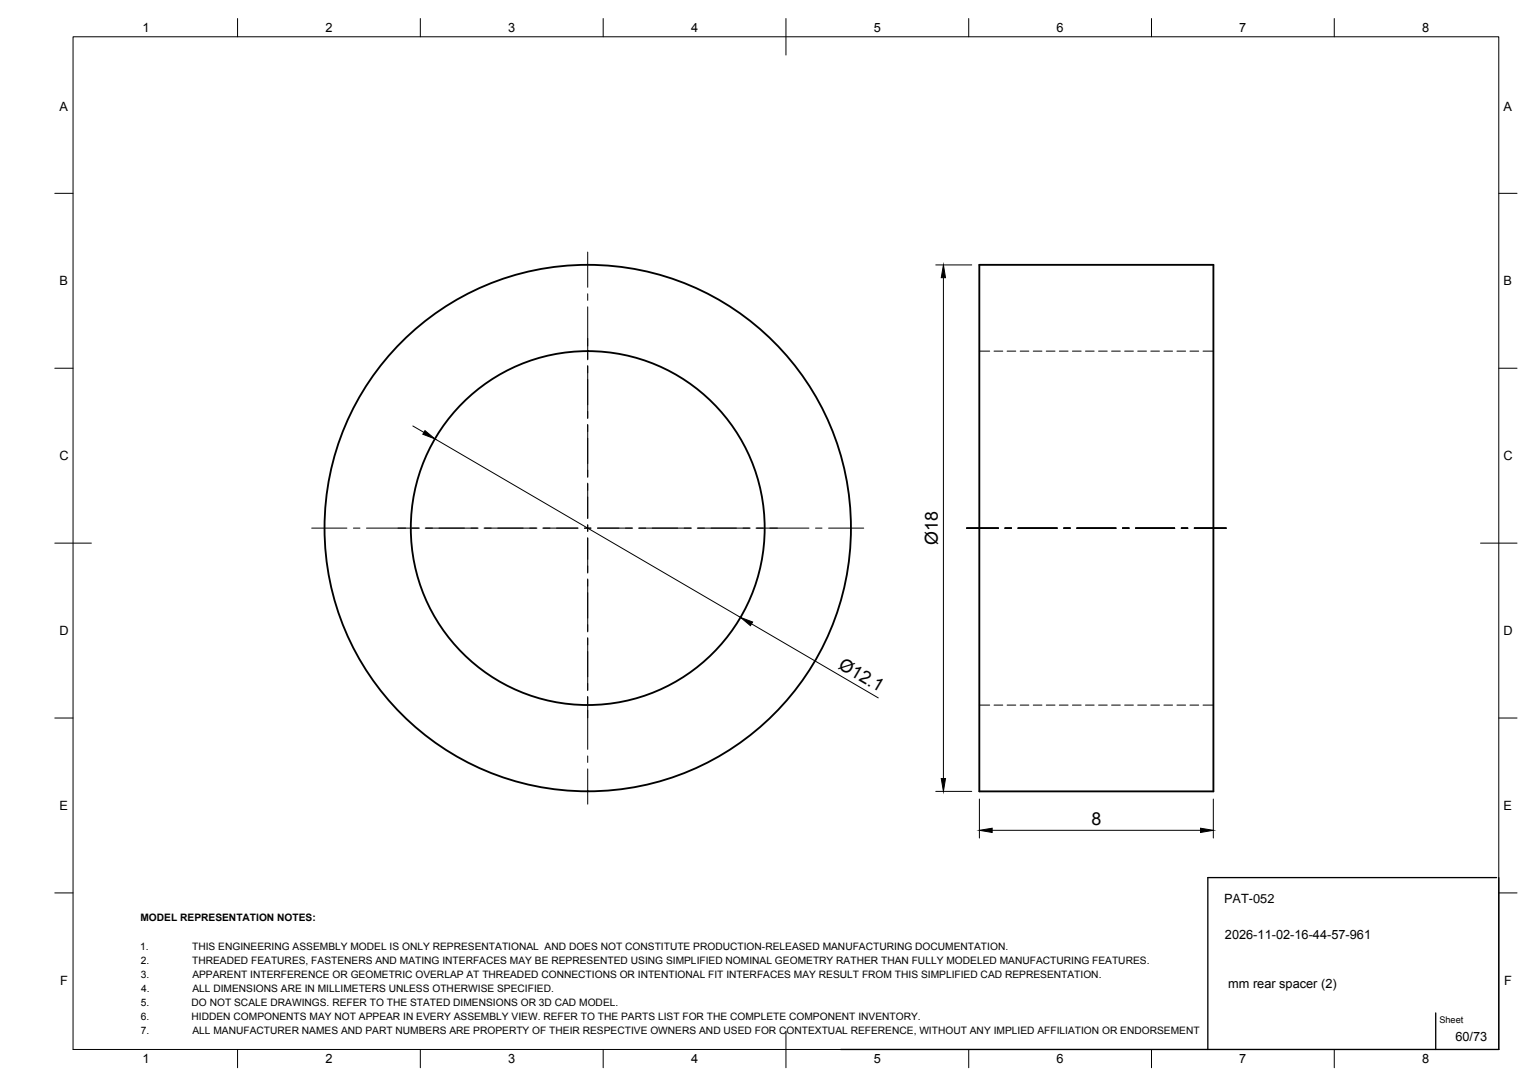
ISO-10303-21;
HEADER;
/* Generated by software containing ST-Developer
 * from STEP Tools, Inc. (www.steptools.com) 
 */

FILE_DESCRIPTION(
/* description */ ('Hand-crank gear train demonstrator'),
/* implementation_level */ '2;1');

FILE_NAME(
/* name */ 'mm rear spacer (2).step',
/* time_stamp */ '2026-10-28T03:22:13-07:00',
/* author */ (''),
/* organization */ (''),
/* preprocessor_version */ 'ST-DEVELOPER v20.2',
/* originating_system */ 'Autodesk Translation Framework v15.17.0.0',
/* authorisation */ '');

FILE_SCHEMA (('AUTOMOTIVE_DESIGN { 1 0 10303 214 3 1 1 }'));
ENDSEC;

DATA;
#10=MECHANICAL_DESIGN_GEOMETRIC_PRESENTATION_REPRESENTATION('',(#1250),#62758);
#1107=SHAPE_REPRESENTATION_RELATIONSHIP('SRR','None',#63084,#1171);
#1171=ADVANCED_BREP_SHAPE_REPRESENTATION('',(#1325),#62738);
#1250=STYLED_ITEM('',(#63476),#1325);
#1325=MANIFOLD_SOLID_BREP('Body1',#16434);
#1592=FACE_BOUND('',#3872,.T.);
#1593=FACE_BOUND('',#3874,.T.);
#1969=PLANE('',#18245);
#1970=PLANE('',#18246);
#2683=FACE_OUTER_BOUND('',#3869,.T.);
#2684=FACE_OUTER_BOUND('',#3870,.T.);
#2685=FACE_OUTER_BOUND('',#3871,.T.);
#2686=FACE_OUTER_BOUND('',#3873,.T.);
#3869=EDGE_LOOP('',(#13199,#13200,#13201,#13202));
#3870=EDGE_LOOP('',(#13203,#13204,#13205,#13206));
#3871=EDGE_LOOP('',(#13207));
#3872=EDGE_LOOP('',(#13208));
#3873=EDGE_LOOP('',(#13209));
#3874=EDGE_LOOP('',(#13210));
#4971=LINE('',#26665,#6103);
#4972=LINE('',#26671,#6104);
#6103=VECTOR('',#21682,0.605);
#6104=VECTOR('',#21689,0.9);
#7007=CIRCLE('',#18240,0.605);
#7008=CIRCLE('',#18241,0.605);
#7009=CIRCLE('',#18243,0.9);
#7010=CIRCLE('',#18244,0.9);
#8014=VERTEX_POINT('',#26662);
#8015=VERTEX_POINT('',#26664);
#8016=VERTEX_POINT('',#26668);
#8017=VERTEX_POINT('',#26670);
#9851=EDGE_CURVE('',#8014,#8014,#7007,.T.);
#9852=EDGE_CURVE('',#8014,#8015,#4971,.T.);
#9853=EDGE_CURVE('',#8015,#8015,#7008,.T.);
#9854=EDGE_CURVE('',#8016,#8016,#7009,.T.);
#9855=EDGE_CURVE('',#8016,#8017,#4972,.T.);
#9856=EDGE_CURVE('',#8017,#8017,#7010,.T.);
#13199=ORIENTED_EDGE('',*,*,#9851,.F.);
#13200=ORIENTED_EDGE('',*,*,#9852,.T.);
#13201=ORIENTED_EDGE('',*,*,#9853,.T.);
#13202=ORIENTED_EDGE('',*,*,#9852,.F.);
#13203=ORIENTED_EDGE('',*,*,#9854,.F.);
#13204=ORIENTED_EDGE('',*,*,#9855,.T.);
#13205=ORIENTED_EDGE('',*,*,#9856,.T.);
#13206=ORIENTED_EDGE('',*,*,#9855,.F.);
#13207=ORIENTED_EDGE('',*,*,#9854,.T.);
#13208=ORIENTED_EDGE('',*,*,#9851,.T.);
#13209=ORIENTED_EDGE('',*,*,#9856,.F.);
#13210=ORIENTED_EDGE('',*,*,#9853,.F.);
#15337=CYLINDRICAL_SURFACE('',#18239,0.605);
#15338=CYLINDRICAL_SURFACE('',#18242,0.9);
#15993=ADVANCED_FACE('',(#2683),#15337,.F.);
#15994=ADVANCED_FACE('',(#2684),#15338,.T.);
#15995=ADVANCED_FACE('',(#2685,#1592),#1969,.T.);
#15996=ADVANCED_FACE('',(#2686,#1593),#1970,.F.);
#16434=CLOSED_SHELL('',(#15993,#15994,#15995,#15996));
#18238=AXIS2_PLACEMENT_3D('',#26660,#21676,#21677);
#18239=AXIS2_PLACEMENT_3D('',#26661,#21678,#21679);
#18240=AXIS2_PLACEMENT_3D('',#26663,#21680,#21681);
#18241=AXIS2_PLACEMENT_3D('',#26666,#21683,#21684);
#18242=AXIS2_PLACEMENT_3D('',#26667,#21685,#21686);
#18243=AXIS2_PLACEMENT_3D('',#26669,#21687,#21688);
#18244=AXIS2_PLACEMENT_3D('',#26672,#21690,#21691);
#18245=AXIS2_PLACEMENT_3D('',#26673,#21692,#21693);
#18246=AXIS2_PLACEMENT_3D('',#26674,#21694,#21695);
#21676=DIRECTION('axis',(0.,0.,1.));
#21677=DIRECTION('refdir',(1.,0.,0.));
#21678=DIRECTION('center_axis',(0.,1.,0.));
#21679=DIRECTION('ref_axis',(1.,0.,0.));
#21680=DIRECTION('center_axis',(0.,-1.,0.));
#21681=DIRECTION('ref_axis',(1.,0.,0.));
#21682=DIRECTION('',(0.,-1.,0.));
#21683=DIRECTION('center_axis',(0.,-1.,0.));
#21684=DIRECTION('ref_axis',(1.,0.,0.));
#21685=DIRECTION('center_axis',(0.,1.,0.));
#21686=DIRECTION('ref_axis',(1.,0.,0.));
#21687=DIRECTION('center_axis',(0.,1.,0.));
#21688=DIRECTION('ref_axis',(1.,0.,0.));
#21689=DIRECTION('',(0.,-1.,0.));
#21690=DIRECTION('center_axis',(0.,1.,0.));
#21691=DIRECTION('ref_axis',(1.,0.,0.));
#21692=DIRECTION('center_axis',(0.,1.,0.));
#21693=DIRECTION('ref_axis',(1.,0.,0.));
#21694=DIRECTION('center_axis',(0.,1.,0.));
#21695=DIRECTION('ref_axis',(1.,0.,0.));
#26660=CARTESIAN_POINT('',(0.,0.,0.));
#26661=CARTESIAN_POINT('Origin',(12.,-2.8,9.));
#26662=CARTESIAN_POINT('',(11.395,-2.,9.));
#26663=CARTESIAN_POINT('Origin',(12.,-2.,9.));
#26664=CARTESIAN_POINT('',(11.395,-2.8,9.));
#26665=CARTESIAN_POINT('',(11.395,-2.8,9.));
#26666=CARTESIAN_POINT('Origin',(12.,-2.8,9.));
#26667=CARTESIAN_POINT('Origin',(12.,-2.8,9.));
#26668=CARTESIAN_POINT('',(11.1,-2.,9.));
#26669=CARTESIAN_POINT('Origin',(12.,-2.,9.));
#26670=CARTESIAN_POINT('',(11.1,-2.8,9.));
#26671=CARTESIAN_POINT('',(11.1,-2.8,9.));
#26672=CARTESIAN_POINT('Origin',(12.,-2.8,9.));
#26673=CARTESIAN_POINT('Origin',(12.,-2.,9.));
#26674=CARTESIAN_POINT('Origin',(12.,-2.8,9.));
#62664=UNCERTAINTY_MEASURE_WITH_UNIT(LENGTH_MEASURE(0.001),#62759,
'DISTANCE_ACCURACY_VALUE',
'Maximum model space distance between geometric entities at asserted c
onnectivities');
#62684=UNCERTAINTY_MEASURE_WITH_UNIT(LENGTH_MEASURE(0.001),#62759,
'DISTANCE_ACCURACY_VALUE',
'Maximum model space distance between geometric entities at asserted c
onnectivities');
#62738=(
GEOMETRIC_REPRESENTATION_CONTEXT(3)
GLOBAL_UNCERTAINTY_ASSIGNED_CONTEXT((#62664))
GLOBAL_UNIT_ASSIGNED_CONTEXT((#62759,#62761,#62762))
REPRESENTATION_CONTEXT('','3D')
);
#62758=(
GEOMETRIC_REPRESENTATION_CONTEXT(3)
GLOBAL_UNCERTAINTY_ASSIGNED_CONTEXT((#62684))
GLOBAL_UNIT_ASSIGNED_CONTEXT((#62759,#62761,#62762))
REPRESENTATION_CONTEXT('','3D')
);
#62759=(
LENGTH_UNIT()
NAMED_UNIT(*)
SI_UNIT(.CENTI.,.METRE.)
);
#62761=(
NAMED_UNIT(*)
PLANE_ANGLE_UNIT()
SI_UNIT($,.RADIAN.)
);
#62762=(
NAMED_UNIT(*)
SI_UNIT($,.STERADIAN.)
SOLID_ANGLE_UNIT()
);
#62816=SHAPE_DEFINITION_REPRESENTATION(#62899,#63084);
#62899=PRODUCT_DEFINITION_SHAPE('',$,#63158);
#63084=SHAPE_REPRESENTATION('',(#18238),#62738);
#63104=PRODUCT_DEFINITION_CONTEXT('part definition',#63325,'design');
#63158=PRODUCT_DEFINITION('mm rear spacer (2)','mm rear spacer (2)',#63231,
#63104);
#63231=PRODUCT_DEFINITION_FORMATION('',$,#63380);
#63325=APPLICATION_CONTEXT(
'Core Data for Automotive Mechanical Design Process');
#63326=PRODUCT_CONTEXT('part definition',#63325,'mechanical');
#63380=PRODUCT('mm rear spacer (2)','mm rear spacer (2)','mm rear spacer (2)',
(#63326));
#63470=COLOUR_RGB('Off White',0.89,0.88,0.83);
#63471=FILL_AREA_STYLE_COLOUR('',#63470);
#63472=FILL_AREA_STYLE('',(#63471));
#63473=SURFACE_STYLE_FILL_AREA(#63472);
#63474=SURFACE_SIDE_STYLE('',(#63473));
#63475=SURFACE_STYLE_USAGE(.BOTH.,#63474);
#63476=PRESENTATION_STYLE_ASSIGNMENT((#63475));
ENDSEC;
END-ISO-10303-21;
